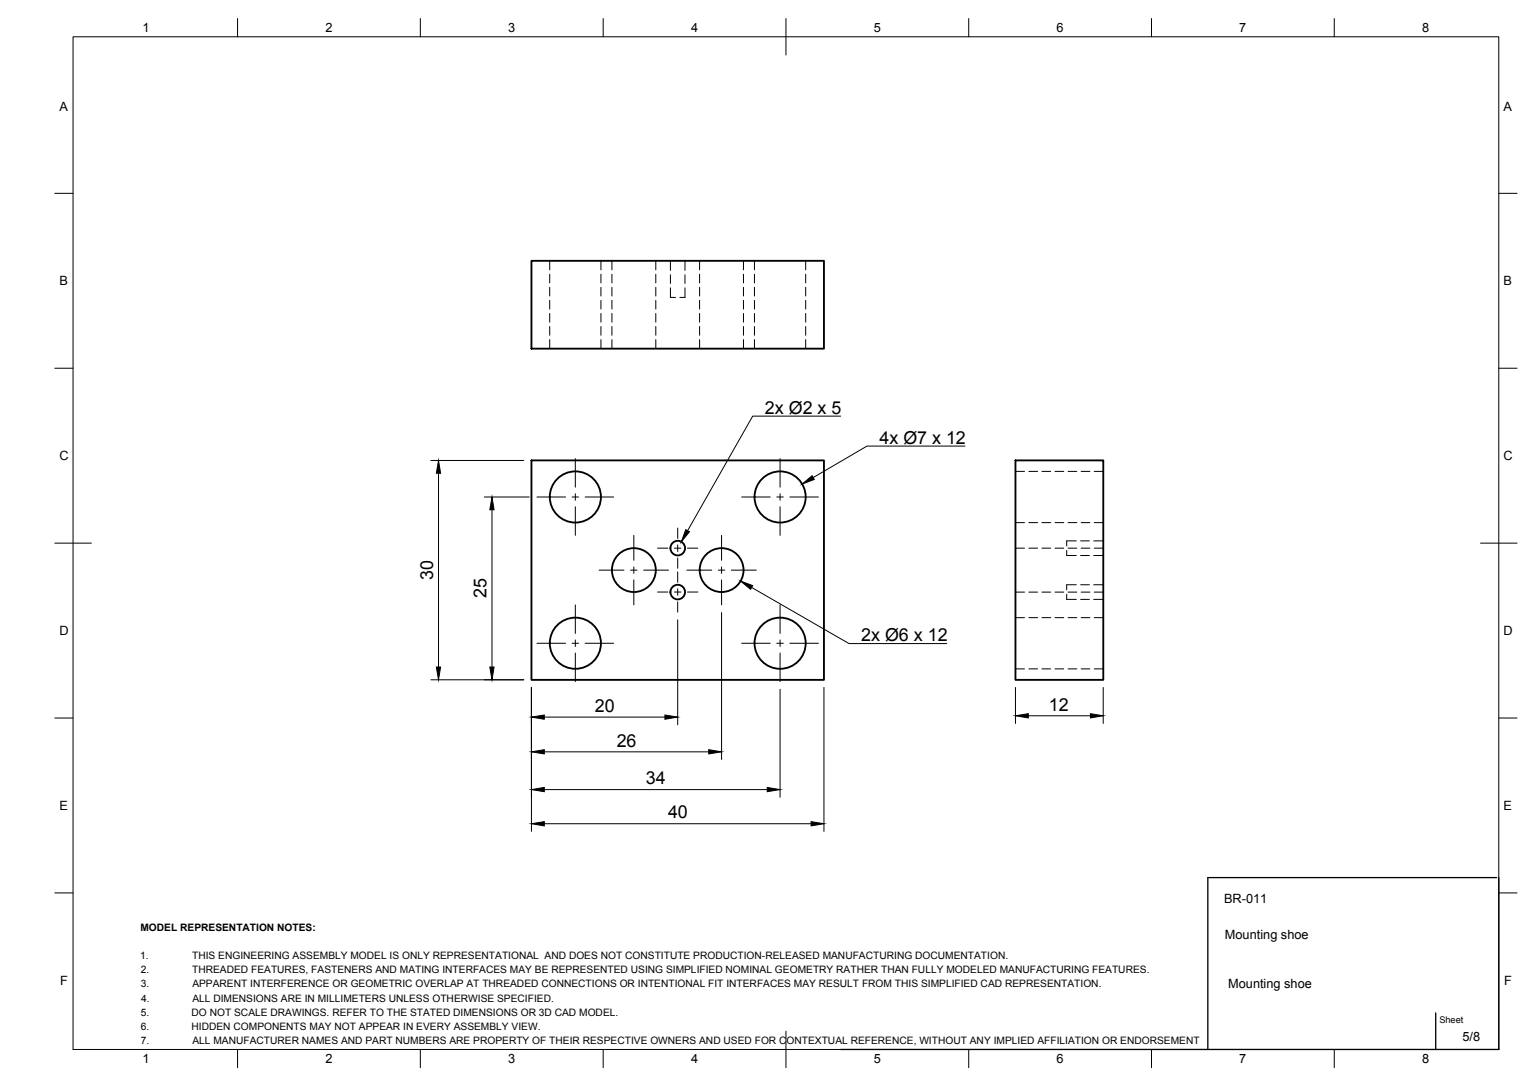
ISO-10303-21;
HEADER;
/* Generated by software containing ST-Developer
 * from STEP Tools, Inc. (www.steptools.com) 
 */

FILE_DESCRIPTION(
/* description */ ('Independent pair of monolithic parallel-leaf compliant finger modules.
 Shared native part/module instances; external gripper actuator outsid
e scope. Whole-mm geometry,1mm webs,56mm straight span,12mm depth,32mm
 nominal contact gap. Undeformed CAD reference; material condition, el
astic range, fatigue and gripping force unassigned.'),
/* implementation_level */ '2;1');

FILE_NAME(
/* name */ 'Mounting shoe.step',
/* time_stamp */ '2026-11-07T22:36:16-08:00',
/* author */ (''),
/* organization */ (''),
/* preprocessor_version */ 'ST-DEVELOPER v20.2',
/* originating_system */ 'Autodesk Translation Framework v15.17.0.0',
/* authorisation */ '');

FILE_SCHEMA (('AUTOMOTIVE_DESIGN { 1 0 10303 214 3 1 1 }'));
ENDSEC;

DATA;
#10=MECHANICAL_DESIGN_GEOMETRIC_PRESENTATION_REPRESENTATION('',(#329),#13801);
#317=SHAPE_REPRESENTATION_RELATIONSHIP('SRR','None',#13835,#323);
#323=ADVANCED_BREP_SHAPE_REPRESENTATION('',(#335),#13795);
#329=STYLED_ITEM('',(#13878),#335);
#335=MANIFOLD_SOLID_BREP('Body1',#3694);
#341=FACE_BOUND('',#630,.T.);
#342=FACE_BOUND('',#631,.T.);
#343=FACE_BOUND('',#632,.T.);
#344=FACE_BOUND('',#633,.T.);
#345=FACE_BOUND('',#634,.T.);
#346=FACE_BOUND('',#635,.T.);
#347=FACE_BOUND('',#636,.T.);
#348=FACE_BOUND('',#637,.T.);
#349=FACE_BOUND('',#640,.T.);
#350=FACE_BOUND('',#641,.T.);
#351=FACE_BOUND('',#642,.T.);
#352=FACE_BOUND('',#643,.T.);
#353=FACE_BOUND('',#644,.T.);
#354=FACE_BOUND('',#645,.T.);
#365=PLANE('',#3773);
#366=PLANE('',#3777);
#367=PLANE('',#3796);
#368=PLANE('',#3797);
#369=PLANE('',#3798);
#370=PLANE('',#3799);
#371=PLANE('',#3800);
#372=PLANE('',#3801);
#417=FACE_OUTER_BOUND('',#618,.T.);
#418=FACE_OUTER_BOUND('',#619,.T.);
#419=FACE_OUTER_BOUND('',#620,.T.);
#420=FACE_OUTER_BOUND('',#621,.T.);
#421=FACE_OUTER_BOUND('',#622,.T.);
#422=FACE_OUTER_BOUND('',#623,.T.);
#423=FACE_OUTER_BOUND('',#624,.T.);
#424=FACE_OUTER_BOUND('',#625,.T.);
#425=FACE_OUTER_BOUND('',#626,.T.);
#426=FACE_OUTER_BOUND('',#627,.T.);
#427=FACE_OUTER_BOUND('',#628,.T.);
#428=FACE_OUTER_BOUND('',#629,.T.);
#429=FACE_OUTER_BOUND('',#638,.T.);
#430=FACE_OUTER_BOUND('',#639,.T.);
#431=FACE_OUTER_BOUND('',#646,.T.);
#432=FACE_OUTER_BOUND('',#647,.T.);
#618=EDGE_LOOP('',(#2265,#2266,#2267,#2268));
#619=EDGE_LOOP('',(#2269));
#620=EDGE_LOOP('',(#2270,#2271,#2272,#2273));
#621=EDGE_LOOP('',(#2274));
#622=EDGE_LOOP('',(#2275,#2276,#2277,#2278));
#623=EDGE_LOOP('',(#2279,#2280,#2281,#2282));
#624=EDGE_LOOP('',(#2283,#2284,#2285,#2286));
#625=EDGE_LOOP('',(#2287,#2288,#2289,#2290));
#626=EDGE_LOOP('',(#2291,#2292,#2293,#2294));
#627=EDGE_LOOP('',(#2295,#2296,#2297,#2298));
#628=EDGE_LOOP('',(#2299,#2300,#2301,#2302));
#629=EDGE_LOOP('',(#2303,#2304,#2305,#2306));
#630=EDGE_LOOP('',(#2307));
#631=EDGE_LOOP('',(#2308));
#632=EDGE_LOOP('',(#2309));
#633=EDGE_LOOP('',(#2310));
#634=EDGE_LOOP('',(#2311));
#635=EDGE_LOOP('',(#2312));
#636=EDGE_LOOP('',(#2313));
#637=EDGE_LOOP('',(#2314));
#638=EDGE_LOOP('',(#2315,#2316,#2317,#2318));
#639=EDGE_LOOP('',(#2319,#2320,#2321,#2322));
#640=EDGE_LOOP('',(#2323));
#641=EDGE_LOOP('',(#2324));
#642=EDGE_LOOP('',(#2325));
#643=EDGE_LOOP('',(#2326));
#644=EDGE_LOOP('',(#2327));
#645=EDGE_LOOP('',(#2328));
#646=EDGE_LOOP('',(#2329,#2330,#2331,#2332));
#647=EDGE_LOOP('',(#2333,#2334,#2335,#2336));
#843=LINE('',#4822,#1072);
#844=LINE('',#4829,#1073);
#845=LINE('',#4836,#1074);
#846=LINE('',#4842,#1075);
#847=LINE('',#4848,#1076);
#848=LINE('',#4854,#1077);
#849=LINE('',#4860,#1078);
#850=LINE('',#4866,#1079);
#851=LINE('',#4871,#1080);
#852=LINE('',#4873,#1081);
#853=LINE('',#4875,#1082);
#854=LINE('',#4876,#1083);
#855=LINE('',#4879,#1084);
#856=LINE('',#4881,#1085);
#857=LINE('',#4882,#1086);
#858=LINE('',#4885,#1087);
#859=LINE('',#4887,#1088);
#860=LINE('',#4888,#1089);
#861=LINE('',#4890,#1090);
#862=LINE('',#4891,#1091);
#1072=VECTOR('',#4050,1.);
#1073=VECTOR('',#4059,1.);
#1074=VECTOR('',#4068,3.5);
#1075=VECTOR('',#4075,3.5);
#1076=VECTOR('',#4082,3.5);
#1077=VECTOR('',#4089,3.5);
#1078=VECTOR('',#4096,3.);
#1079=VECTOR('',#4103,3.);
#1080=VECTOR('',#4108,10.);
#1081=VECTOR('',#4109,10.);
#1082=VECTOR('',#4110,10.);
#1083=VECTOR('',#4111,10.);
#1084=VECTOR('',#4114,10.);
#1085=VECTOR('',#4115,10.);
#1086=VECTOR('',#4116,10.);
#1087=VECTOR('',#4119,10.);
#1088=VECTOR('',#4120,10.);
#1089=VECTOR('',#4121,10.);
#1090=VECTOR('',#4124,10.);
#1091=VECTOR('',#4125,10.);
#1301=CIRCLE('',#3771,1.);
#1302=CIRCLE('',#3772,1.);
#1303=CIRCLE('',#3775,1.);
#1304=CIRCLE('',#3776,1.);
#1305=CIRCLE('',#3779,3.5);
#1306=CIRCLE('',#3780,3.5);
#1307=CIRCLE('',#3782,3.5);
#1308=CIRCLE('',#3783,3.5);
#1309=CIRCLE('',#3785,3.5);
#1310=CIRCLE('',#3786,3.5);
#1311=CIRCLE('',#3788,3.5);
#1312=CIRCLE('',#3789,3.5);
#1313=CIRCLE('',#3791,3.);
#1314=CIRCLE('',#3792,3.);
#1315=CIRCLE('',#3794,3.);
#1316=CIRCLE('',#3795,3.);
#1360=VERTEX_POINT('',#4819);
#1361=VERTEX_POINT('',#4821);
#1362=VERTEX_POINT('',#4826);
#1363=VERTEX_POINT('',#4828);
#1364=VERTEX_POINT('',#4833);
#1365=VERTEX_POINT('',#4835);
#1366=VERTEX_POINT('',#4839);
#1367=VERTEX_POINT('',#4841);
#1368=VERTEX_POINT('',#4845);
#1369=VERTEX_POINT('',#4847);
#1370=VERTEX_POINT('',#4851);
#1371=VERTEX_POINT('',#4853);
#1372=VERTEX_POINT('',#4857);
#1373=VERTEX_POINT('',#4859);
#1374=VERTEX_POINT('',#4863);
#1375=VERTEX_POINT('',#4865);
#1376=VERTEX_POINT('',#4869);
#1377=VERTEX_POINT('',#4870);
#1378=VERTEX_POINT('',#4872);
#1379=VERTEX_POINT('',#4874);
#1380=VERTEX_POINT('',#4878);
#1381=VERTEX_POINT('',#4880);
#1382=VERTEX_POINT('',#4884);
#1383=VERTEX_POINT('',#4886);
#1722=EDGE_CURVE('',#1360,#1360,#1301,.T.);
#1723=EDGE_CURVE('',#1360,#1361,#843,.T.);
#1724=EDGE_CURVE('',#1361,#1361,#1302,.T.);
#1725=EDGE_CURVE('',#1362,#1362,#1303,.T.);
#1726=EDGE_CURVE('',#1362,#1363,#844,.T.);
#1727=EDGE_CURVE('',#1363,#1363,#1304,.T.);
#1728=EDGE_CURVE('',#1364,#1364,#1305,.T.);
#1729=EDGE_CURVE('',#1364,#1365,#845,.T.);
#1730=EDGE_CURVE('',#1365,#1365,#1306,.T.);
#1731=EDGE_CURVE('',#1366,#1366,#1307,.T.);
#1732=EDGE_CURVE('',#1366,#1367,#846,.T.);
#1733=EDGE_CURVE('',#1367,#1367,#1308,.T.);
#1734=EDGE_CURVE('',#1368,#1368,#1309,.T.);
#1735=EDGE_CURVE('',#1368,#1369,#847,.T.);
#1736=EDGE_CURVE('',#1369,#1369,#1310,.T.);
#1737=EDGE_CURVE('',#1370,#1370,#1311,.T.);
#1738=EDGE_CURVE('',#1370,#1371,#848,.T.);
#1739=EDGE_CURVE('',#1371,#1371,#1312,.T.);
#1740=EDGE_CURVE('',#1372,#1372,#1313,.T.);
#1741=EDGE_CURVE('',#1372,#1373,#849,.T.);
#1742=EDGE_CURVE('',#1373,#1373,#1314,.T.);
#1743=EDGE_CURVE('',#1374,#1374,#1315,.T.);
#1744=EDGE_CURVE('',#1374,#1375,#850,.T.);
#1745=EDGE_CURVE('',#1375,#1375,#1316,.T.);
#1746=EDGE_CURVE('',#1376,#1377,#851,.T.);
#1747=EDGE_CURVE('',#1377,#1378,#852,.T.);
#1748=EDGE_CURVE('',#1379,#1378,#853,.T.);
#1749=EDGE_CURVE('',#1376,#1379,#854,.T.);
#1750=EDGE_CURVE('',#1380,#1376,#855,.T.);
#1751=EDGE_CURVE('',#1381,#1379,#856,.T.);
#1752=EDGE_CURVE('',#1380,#1381,#857,.T.);
#1753=EDGE_CURVE('',#1382,#1380,#858,.T.);
#1754=EDGE_CURVE('',#1383,#1381,#859,.T.);
#1755=EDGE_CURVE('',#1382,#1383,#860,.T.);
#1756=EDGE_CURVE('',#1377,#1382,#861,.T.);
#1757=EDGE_CURVE('',#1378,#1383,#862,.T.);
#2265=ORIENTED_EDGE('',*,*,#1722,.F.);
#2266=ORIENTED_EDGE('',*,*,#1723,.T.);
#2267=ORIENTED_EDGE('',*,*,#1724,.T.);
#2268=ORIENTED_EDGE('',*,*,#1723,.F.);
#2269=ORIENTED_EDGE('',*,*,#1724,.F.);
#2270=ORIENTED_EDGE('',*,*,#1725,.F.);
#2271=ORIENTED_EDGE('',*,*,#1726,.T.);
#2272=ORIENTED_EDGE('',*,*,#1727,.T.);
#2273=ORIENTED_EDGE('',*,*,#1726,.F.);
#2274=ORIENTED_EDGE('',*,*,#1727,.F.);
#2275=ORIENTED_EDGE('',*,*,#1728,.F.);
#2276=ORIENTED_EDGE('',*,*,#1729,.T.);
#2277=ORIENTED_EDGE('',*,*,#1730,.F.);
#2278=ORIENTED_EDGE('',*,*,#1729,.F.);
#2279=ORIENTED_EDGE('',*,*,#1731,.F.);
#2280=ORIENTED_EDGE('',*,*,#1732,.T.);
#2281=ORIENTED_EDGE('',*,*,#1733,.F.);
#2282=ORIENTED_EDGE('',*,*,#1732,.F.);
#2283=ORIENTED_EDGE('',*,*,#1734,.F.);
#2284=ORIENTED_EDGE('',*,*,#1735,.T.);
#2285=ORIENTED_EDGE('',*,*,#1736,.F.);
#2286=ORIENTED_EDGE('',*,*,#1735,.F.);
#2287=ORIENTED_EDGE('',*,*,#1737,.F.);
#2288=ORIENTED_EDGE('',*,*,#1738,.T.);
#2289=ORIENTED_EDGE('',*,*,#1739,.F.);
#2290=ORIENTED_EDGE('',*,*,#1738,.F.);
#2291=ORIENTED_EDGE('',*,*,#1740,.F.);
#2292=ORIENTED_EDGE('',*,*,#1741,.T.);
#2293=ORIENTED_EDGE('',*,*,#1742,.F.);
#2294=ORIENTED_EDGE('',*,*,#1741,.F.);
#2295=ORIENTED_EDGE('',*,*,#1743,.F.);
#2296=ORIENTED_EDGE('',*,*,#1744,.T.);
#2297=ORIENTED_EDGE('',*,*,#1745,.F.);
#2298=ORIENTED_EDGE('',*,*,#1744,.F.);
#2299=ORIENTED_EDGE('',*,*,#1746,.T.);
#2300=ORIENTED_EDGE('',*,*,#1747,.T.);
#2301=ORIENTED_EDGE('',*,*,#1748,.F.);
#2302=ORIENTED_EDGE('',*,*,#1749,.F.);
#2303=ORIENTED_EDGE('',*,*,#1750,.T.);
#2304=ORIENTED_EDGE('',*,*,#1749,.T.);
#2305=ORIENTED_EDGE('',*,*,#1751,.F.);
#2306=ORIENTED_EDGE('',*,*,#1752,.F.);
#2307=ORIENTED_EDGE('',*,*,#1730,.T.);
#2308=ORIENTED_EDGE('',*,*,#1733,.T.);
#2309=ORIENTED_EDGE('',*,*,#1736,.T.);
#2310=ORIENTED_EDGE('',*,*,#1739,.T.);
#2311=ORIENTED_EDGE('',*,*,#1742,.T.);
#2312=ORIENTED_EDGE('',*,*,#1745,.T.);
#2313=ORIENTED_EDGE('',*,*,#1725,.T.);
#2314=ORIENTED_EDGE('',*,*,#1722,.T.);
#2315=ORIENTED_EDGE('',*,*,#1753,.T.);
#2316=ORIENTED_EDGE('',*,*,#1752,.T.);
#2317=ORIENTED_EDGE('',*,*,#1754,.F.);
#2318=ORIENTED_EDGE('',*,*,#1755,.F.);
#2319=ORIENTED_EDGE('',*,*,#1756,.T.);
#2320=ORIENTED_EDGE('',*,*,#1755,.T.);
#2321=ORIENTED_EDGE('',*,*,#1757,.F.);
#2322=ORIENTED_EDGE('',*,*,#1747,.F.);
#2323=ORIENTED_EDGE('',*,*,#1743,.T.);
#2324=ORIENTED_EDGE('',*,*,#1740,.T.);
#2325=ORIENTED_EDGE('',*,*,#1737,.T.);
#2326=ORIENTED_EDGE('',*,*,#1734,.T.);
#2327=ORIENTED_EDGE('',*,*,#1731,.T.);
#2328=ORIENTED_EDGE('',*,*,#1728,.T.);
#2329=ORIENTED_EDGE('',*,*,#1757,.T.);
#2330=ORIENTED_EDGE('',*,*,#1754,.T.);
#2331=ORIENTED_EDGE('',*,*,#1751,.T.);
#2332=ORIENTED_EDGE('',*,*,#1748,.T.);
#2333=ORIENTED_EDGE('',*,*,#1756,.F.);
#2334=ORIENTED_EDGE('',*,*,#1746,.F.);
#2335=ORIENTED_EDGE('',*,*,#1750,.F.);
#2336=ORIENTED_EDGE('',*,*,#1753,.F.);
#3351=CYLINDRICAL_SURFACE('',#3770,1.);
#3352=CYLINDRICAL_SURFACE('',#3774,1.);
#3353=CYLINDRICAL_SURFACE('',#3778,3.5);
#3354=CYLINDRICAL_SURFACE('',#3781,3.5);
#3355=CYLINDRICAL_SURFACE('',#3784,3.5);
#3356=CYLINDRICAL_SURFACE('',#3787,3.5);
#3357=CYLINDRICAL_SURFACE('',#3790,3.);
#3358=CYLINDRICAL_SURFACE('',#3793,3.);
#3493=ADVANCED_FACE('',(#417),#3351,.F.);
#3494=ADVANCED_FACE('',(#418),#365,.F.);
#3495=ADVANCED_FACE('',(#419),#3352,.F.);
#3496=ADVANCED_FACE('',(#420),#366,.F.);
#3497=ADVANCED_FACE('',(#421),#3353,.F.);
#3498=ADVANCED_FACE('',(#422),#3354,.F.);
#3499=ADVANCED_FACE('',(#423),#3355,.F.);
#3500=ADVANCED_FACE('',(#424),#3356,.F.);
#3501=ADVANCED_FACE('',(#425),#3357,.F.);
#3502=ADVANCED_FACE('',(#426),#3358,.F.);
#3503=ADVANCED_FACE('',(#427),#367,.T.);
#3504=ADVANCED_FACE('',(#428,#341,#342,#343,#344,#345,#346,#347,#348),#368,
 .T.);
#3505=ADVANCED_FACE('',(#429),#369,.T.);
#3506=ADVANCED_FACE('',(#430,#349,#350,#351,#352,#353,#354),#370,.T.);
#3507=ADVANCED_FACE('',(#431),#371,.T.);
#3508=ADVANCED_FACE('',(#432),#372,.F.);
#3694=CLOSED_SHELL('',(#3493,#3494,#3495,#3496,#3497,#3498,#3499,#3500,
#3501,#3502,#3503,#3504,#3505,#3506,#3507,#3508));
#3769=AXIS2_PLACEMENT_3D('',#4817,#4044,#4045);
#3770=AXIS2_PLACEMENT_3D('',#4818,#4046,#4047);
#3771=AXIS2_PLACEMENT_3D('',#4820,#4048,#4049);
#3772=AXIS2_PLACEMENT_3D('',#4823,#4051,#4052);
#3773=AXIS2_PLACEMENT_3D('',#4824,#4053,#4054);
#3774=AXIS2_PLACEMENT_3D('',#4825,#4055,#4056);
#3775=AXIS2_PLACEMENT_3D('',#4827,#4057,#4058);
#3776=AXIS2_PLACEMENT_3D('',#4830,#4060,#4061);
#3777=AXIS2_PLACEMENT_3D('',#4831,#4062,#4063);
#3778=AXIS2_PLACEMENT_3D('',#4832,#4064,#4065);
#3779=AXIS2_PLACEMENT_3D('',#4834,#4066,#4067);
#3780=AXIS2_PLACEMENT_3D('',#4837,#4069,#4070);
#3781=AXIS2_PLACEMENT_3D('',#4838,#4071,#4072);
#3782=AXIS2_PLACEMENT_3D('',#4840,#4073,#4074);
#3783=AXIS2_PLACEMENT_3D('',#4843,#4076,#4077);
#3784=AXIS2_PLACEMENT_3D('',#4844,#4078,#4079);
#3785=AXIS2_PLACEMENT_3D('',#4846,#4080,#4081);
#3786=AXIS2_PLACEMENT_3D('',#4849,#4083,#4084);
#3787=AXIS2_PLACEMENT_3D('',#4850,#4085,#4086);
#3788=AXIS2_PLACEMENT_3D('',#4852,#4087,#4088);
#3789=AXIS2_PLACEMENT_3D('',#4855,#4090,#4091);
#3790=AXIS2_PLACEMENT_3D('',#4856,#4092,#4093);
#3791=AXIS2_PLACEMENT_3D('',#4858,#4094,#4095);
#3792=AXIS2_PLACEMENT_3D('',#4861,#4097,#4098);
#3793=AXIS2_PLACEMENT_3D('',#4862,#4099,#4100);
#3794=AXIS2_PLACEMENT_3D('',#4864,#4101,#4102);
#3795=AXIS2_PLACEMENT_3D('',#4867,#4104,#4105);
#3796=AXIS2_PLACEMENT_3D('',#4868,#4106,#4107);
#3797=AXIS2_PLACEMENT_3D('',#4877,#4112,#4113);
#3798=AXIS2_PLACEMENT_3D('',#4883,#4117,#4118);
#3799=AXIS2_PLACEMENT_3D('',#4889,#4122,#4123);
#3800=AXIS2_PLACEMENT_3D('',#4892,#4126,#4127);
#3801=AXIS2_PLACEMENT_3D('',#4893,#4128,#4129);
#4044=DIRECTION('axis',(0.,0.,1.));
#4045=DIRECTION('refdir',(1.,0.,0.));
#4046=DIRECTION('center_axis',(-1.,0.,0.));
#4047=DIRECTION('ref_axis',(0.,1.,0.));
#4048=DIRECTION('center_axis',(-1.,0.,0.));
#4049=DIRECTION('ref_axis',(0.,1.,0.));
#4050=DIRECTION('',(-1.,0.,0.));
#4051=DIRECTION('center_axis',(-1.,0.,0.));
#4052=DIRECTION('ref_axis',(0.,1.,0.));
#4053=DIRECTION('center_axis',(-1.,0.,0.));
#4054=DIRECTION('ref_axis',(0.,1.,0.));
#4055=DIRECTION('center_axis',(-1.,0.,0.));
#4056=DIRECTION('ref_axis',(0.,1.,0.));
#4057=DIRECTION('center_axis',(-1.,0.,0.));
#4058=DIRECTION('ref_axis',(0.,1.,0.));
#4059=DIRECTION('',(-1.,0.,0.));
#4060=DIRECTION('center_axis',(-1.,0.,0.));
#4061=DIRECTION('ref_axis',(0.,1.,0.));
#4062=DIRECTION('center_axis',(-1.,0.,0.));
#4063=DIRECTION('ref_axis',(0.,1.,0.));
#4064=DIRECTION('center_axis',(1.,0.,0.));
#4065=DIRECTION('ref_axis',(0.,-1.,0.));
#4066=DIRECTION('center_axis',(1.,0.,0.));
#4067=DIRECTION('ref_axis',(0.,-1.,0.));
#4068=DIRECTION('',(1.,0.,0.));
#4069=DIRECTION('center_axis',(-1.,0.,0.));
#4070=DIRECTION('ref_axis',(0.,-1.,0.));
#4071=DIRECTION('center_axis',(1.,0.,0.));
#4072=DIRECTION('ref_axis',(0.,-1.,0.));
#4073=DIRECTION('center_axis',(1.,0.,0.));
#4074=DIRECTION('ref_axis',(0.,-1.,0.));
#4075=DIRECTION('',(1.,0.,0.));
#4076=DIRECTION('center_axis',(-1.,0.,0.));
#4077=DIRECTION('ref_axis',(0.,-1.,0.));
#4078=DIRECTION('center_axis',(1.,0.,0.));
#4079=DIRECTION('ref_axis',(0.,-1.,0.));
#4080=DIRECTION('center_axis',(1.,0.,0.));
#4081=DIRECTION('ref_axis',(0.,-1.,0.));
#4082=DIRECTION('',(1.,0.,0.));
#4083=DIRECTION('center_axis',(-1.,0.,0.));
#4084=DIRECTION('ref_axis',(0.,-1.,0.));
#4085=DIRECTION('center_axis',(1.,0.,0.));
#4086=DIRECTION('ref_axis',(0.,-1.,0.));
#4087=DIRECTION('center_axis',(1.,0.,0.));
#4088=DIRECTION('ref_axis',(0.,-1.,0.));
#4089=DIRECTION('',(1.,0.,0.));
#4090=DIRECTION('center_axis',(-1.,0.,0.));
#4091=DIRECTION('ref_axis',(0.,-1.,0.));
#4092=DIRECTION('center_axis',(1.,0.,0.));
#4093=DIRECTION('ref_axis',(0.,-1.,0.));
#4094=DIRECTION('center_axis',(1.,0.,0.));
#4095=DIRECTION('ref_axis',(0.,-1.,0.));
#4096=DIRECTION('',(1.,0.,0.));
#4097=DIRECTION('center_axis',(-1.,0.,0.));
#4098=DIRECTION('ref_axis',(0.,-1.,0.));
#4099=DIRECTION('center_axis',(1.,0.,0.));
#4100=DIRECTION('ref_axis',(0.,-1.,0.));
#4101=DIRECTION('center_axis',(1.,0.,0.));
#4102=DIRECTION('ref_axis',(0.,-1.,0.));
#4103=DIRECTION('',(1.,0.,0.));
#4104=DIRECTION('center_axis',(-1.,0.,0.));
#4105=DIRECTION('ref_axis',(0.,-1.,0.));
#4106=DIRECTION('center_axis',(0.,1.,0.));
#4107=DIRECTION('ref_axis',(-1.,0.,0.));
#4108=DIRECTION('',(-1.,0.,0.));
#4109=DIRECTION('',(0.,0.,1.));
#4110=DIRECTION('',(-1.,0.,0.));
#4111=DIRECTION('',(0.,0.,1.));
#4112=DIRECTION('center_axis',(1.,0.,0.));
#4113=DIRECTION('ref_axis',(0.,1.,0.));
#4114=DIRECTION('',(0.,1.,0.));
#4115=DIRECTION('',(0.,1.,0.));
#4116=DIRECTION('',(0.,0.,1.));
#4117=DIRECTION('center_axis',(0.,-1.,0.));
#4118=DIRECTION('ref_axis',(1.,0.,0.));
#4119=DIRECTION('',(1.,0.,0.));
#4120=DIRECTION('',(1.,0.,0.));
#4121=DIRECTION('',(0.,0.,1.));
#4122=DIRECTION('center_axis',(-1.,0.,0.));
#4123=DIRECTION('ref_axis',(0.,-1.,0.));
#4124=DIRECTION('',(0.,-1.,0.));
#4125=DIRECTION('',(0.,-1.,0.));
#4126=DIRECTION('center_axis',(0.,0.,1.));
#4127=DIRECTION('ref_axis',(1.,0.,0.));
#4128=DIRECTION('center_axis',(0.,0.,1.));
#4129=DIRECTION('ref_axis',(1.,0.,0.));
#4817=CARTESIAN_POINT('',(0.,0.,0.));
#4818=CARTESIAN_POINT('Origin',(-2.5,0.,-3.));
#4819=CARTESIAN_POINT('',(0.,-1.,-3.));
#4820=CARTESIAN_POINT('Origin',(0.,0.,-3.));
#4821=CARTESIAN_POINT('',(-5.,-1.,-3.));
#4822=CARTESIAN_POINT('',(-2.5,-1.,-3.));
#4823=CARTESIAN_POINT('Origin',(-5.,0.,-3.));
#4824=CARTESIAN_POINT('Origin',(-5.,0.,-3.));
#4825=CARTESIAN_POINT('Origin',(-2.5,0.,3.));
#4826=CARTESIAN_POINT('',(0.,-1.,3.));
#4827=CARTESIAN_POINT('Origin',(0.,0.,3.));
#4828=CARTESIAN_POINT('',(-5.,-1.,3.));
#4829=CARTESIAN_POINT('',(-2.5,-1.,3.));
#4830=CARTESIAN_POINT('Origin',(-5.,0.,3.));
#4831=CARTESIAN_POINT('Origin',(-5.,0.,3.));
#4832=CARTESIAN_POINT('Origin',(-6.,14.,-10.));
#4833=CARTESIAN_POINT('',(-12.,17.5,-10.));
#4834=CARTESIAN_POINT('Origin',(-12.,14.,-10.));
#4835=CARTESIAN_POINT('',(0.,17.5,-10.));
#4836=CARTESIAN_POINT('',(-6.,17.5,-10.));
#4837=CARTESIAN_POINT('Origin',(0.,14.,-10.));
#4838=CARTESIAN_POINT('Origin',(-6.,-14.,-10.));
#4839=CARTESIAN_POINT('',(-12.,-10.5,-10.));
#4840=CARTESIAN_POINT('Origin',(-12.,-14.,-10.));
#4841=CARTESIAN_POINT('',(0.,-10.5,-10.));
#4842=CARTESIAN_POINT('',(-6.,-10.5,-10.));
#4843=CARTESIAN_POINT('Origin',(0.,-14.,-10.));
#4844=CARTESIAN_POINT('Origin',(-6.,-14.,10.));
#4845=CARTESIAN_POINT('',(-12.,-10.5,10.));
#4846=CARTESIAN_POINT('Origin',(-12.,-14.,10.));
#4847=CARTESIAN_POINT('',(0.,-10.5,10.));
#4848=CARTESIAN_POINT('',(-6.,-10.5,10.));
#4849=CARTESIAN_POINT('Origin',(0.,-14.,10.));
#4850=CARTESIAN_POINT('Origin',(-6.,14.,10.));
#4851=CARTESIAN_POINT('',(-12.,17.5,10.));
#4852=CARTESIAN_POINT('Origin',(-12.,14.,10.));
#4853=CARTESIAN_POINT('',(0.,17.5,10.));
#4854=CARTESIAN_POINT('',(-6.,17.5,10.));
#4855=CARTESIAN_POINT('Origin',(0.,14.,10.));
#4856=CARTESIAN_POINT('Origin',(-6.,-6.,0.));
#4857=CARTESIAN_POINT('',(-12.,-3.,3.67394039744206E-16));
#4858=CARTESIAN_POINT('Origin',(-12.,-6.,0.));
#4859=CARTESIAN_POINT('',(0.,-3.,3.67394039744206E-16));
#4860=CARTESIAN_POINT('',(-6.,-3.,3.67394039744206E-16));
#4861=CARTESIAN_POINT('Origin',(0.,-6.,0.));
#4862=CARTESIAN_POINT('Origin',(-6.,6.,0.));
#4863=CARTESIAN_POINT('',(-12.,9.,3.67394039744206E-16));
#4864=CARTESIAN_POINT('Origin',(-12.,6.,0.));
#4865=CARTESIAN_POINT('',(0.,9.,3.67394039744206E-16));
#4866=CARTESIAN_POINT('',(-6.,9.,3.67394039744206E-16));
#4867=CARTESIAN_POINT('Origin',(0.,6.,0.));
#4868=CARTESIAN_POINT('Origin',(0.,20.,-15.));
#4869=CARTESIAN_POINT('',(0.,20.,-15.));
#4870=CARTESIAN_POINT('',(-12.,20.,-15.));
#4871=CARTESIAN_POINT('',(0.,20.,-15.));
#4872=CARTESIAN_POINT('',(-12.,20.,15.));
#4873=CARTESIAN_POINT('',(-12.,20.,-15.));
#4874=CARTESIAN_POINT('',(0.,20.,15.));
#4875=CARTESIAN_POINT('',(0.,20.,15.));
#4876=CARTESIAN_POINT('',(0.,20.,-15.));
#4877=CARTESIAN_POINT('Origin',(0.,-20.,-15.));
#4878=CARTESIAN_POINT('',(0.,-20.,-15.));
#4879=CARTESIAN_POINT('',(0.,-20.,-15.));
#4880=CARTESIAN_POINT('',(0.,-20.,15.));
#4881=CARTESIAN_POINT('',(0.,-20.,15.));
#4882=CARTESIAN_POINT('',(0.,-20.,-15.));
#4883=CARTESIAN_POINT('Origin',(-12.,-20.,-15.));
#4884=CARTESIAN_POINT('',(-12.,-20.,-15.));
#4885=CARTESIAN_POINT('',(-12.,-20.,-15.));
#4886=CARTESIAN_POINT('',(-12.,-20.,15.));
#4887=CARTESIAN_POINT('',(-12.,-20.,15.));
#4888=CARTESIAN_POINT('',(-12.,-20.,-15.));
#4889=CARTESIAN_POINT('Origin',(-12.,20.,-15.));
#4890=CARTESIAN_POINT('',(-12.,20.,-15.));
#4891=CARTESIAN_POINT('',(-12.,20.,15.));
#4892=CARTESIAN_POINT('Origin',(-6.,0.,15.));
#4893=CARTESIAN_POINT('Origin',(-6.,0.,-15.));
#13786=UNCERTAINTY_MEASURE_WITH_UNIT(LENGTH_MEASURE(0.01),#13802,
'DISTANCE_ACCURACY_VALUE',
'Maximum model space distance between geometric entities at asserted c
onnectivities');
#13792=UNCERTAINTY_MEASURE_WITH_UNIT(LENGTH_MEASURE(0.01),#13802,
'DISTANCE_ACCURACY_VALUE',
'Maximum model space distance between geometric entities at asserted c
onnectivities');
#13795=(
GEOMETRIC_REPRESENTATION_CONTEXT(3)
GLOBAL_UNCERTAINTY_ASSIGNED_CONTEXT((#13786))
GLOBAL_UNIT_ASSIGNED_CONTEXT((#13802,#13804,#13805))
REPRESENTATION_CONTEXT('','3D')
);
#13801=(
GEOMETRIC_REPRESENTATION_CONTEXT(3)
GLOBAL_UNCERTAINTY_ASSIGNED_CONTEXT((#13792))
GLOBAL_UNIT_ASSIGNED_CONTEXT((#13802,#13804,#13805))
REPRESENTATION_CONTEXT('','3D')
);
#13802=(
LENGTH_UNIT()
NAMED_UNIT(*)
SI_UNIT(.MILLI.,.METRE.)
);
#13804=(
NAMED_UNIT(*)
PLANE_ANGLE_UNIT()
SI_UNIT($,.RADIAN.)
);
#13805=(
NAMED_UNIT(*)
SI_UNIT($,.STERADIAN.)
SOLID_ANGLE_UNIT()
);
#13808=SHAPE_DEFINITION_REPRESENTATION(#13816,#13835);
#13816=PRODUCT_DEFINITION_SHAPE('',$,#13844);
#13835=SHAPE_REPRESENTATION('',(#3769),#13795);
#13841=PRODUCT_DEFINITION_CONTEXT('part definition',#13867,'design');
#13844=PRODUCT_DEFINITION('Mounting shoe','Mounting shoe',#13852,#13841);
#13852=PRODUCT_DEFINITION_FORMATION('',$,#13871);
#13867=APPLICATION_CONTEXT(
'Core Data for Automotive Mechanical Design Process');
#13868=PRODUCT_CONTEXT('part definition',#13867,'mechanical');
#13871=PRODUCT('Mounting shoe','Mounting shoe',$,(#13868));
#13878=PRESENTATION_STYLE_ASSIGNMENT((#13885));
#13885=SURFACE_STYLE_USAGE(.BOTH.,#13892);
#13892=SURFACE_SIDE_STYLE('',(#13899));
#13899=SURFACE_STYLE_FILL_AREA(#13906);
#13906=FILL_AREA_STYLE('Dark blue',(#13913));
#13913=FILL_AREA_STYLE_COLOUR('Dark blue',#13920);
#13920=COLOUR_RGB('Dark blue',0.0901960784313725,0.270588235294118,0.513725490196078);
ENDSEC;
END-ISO-10303-21;
